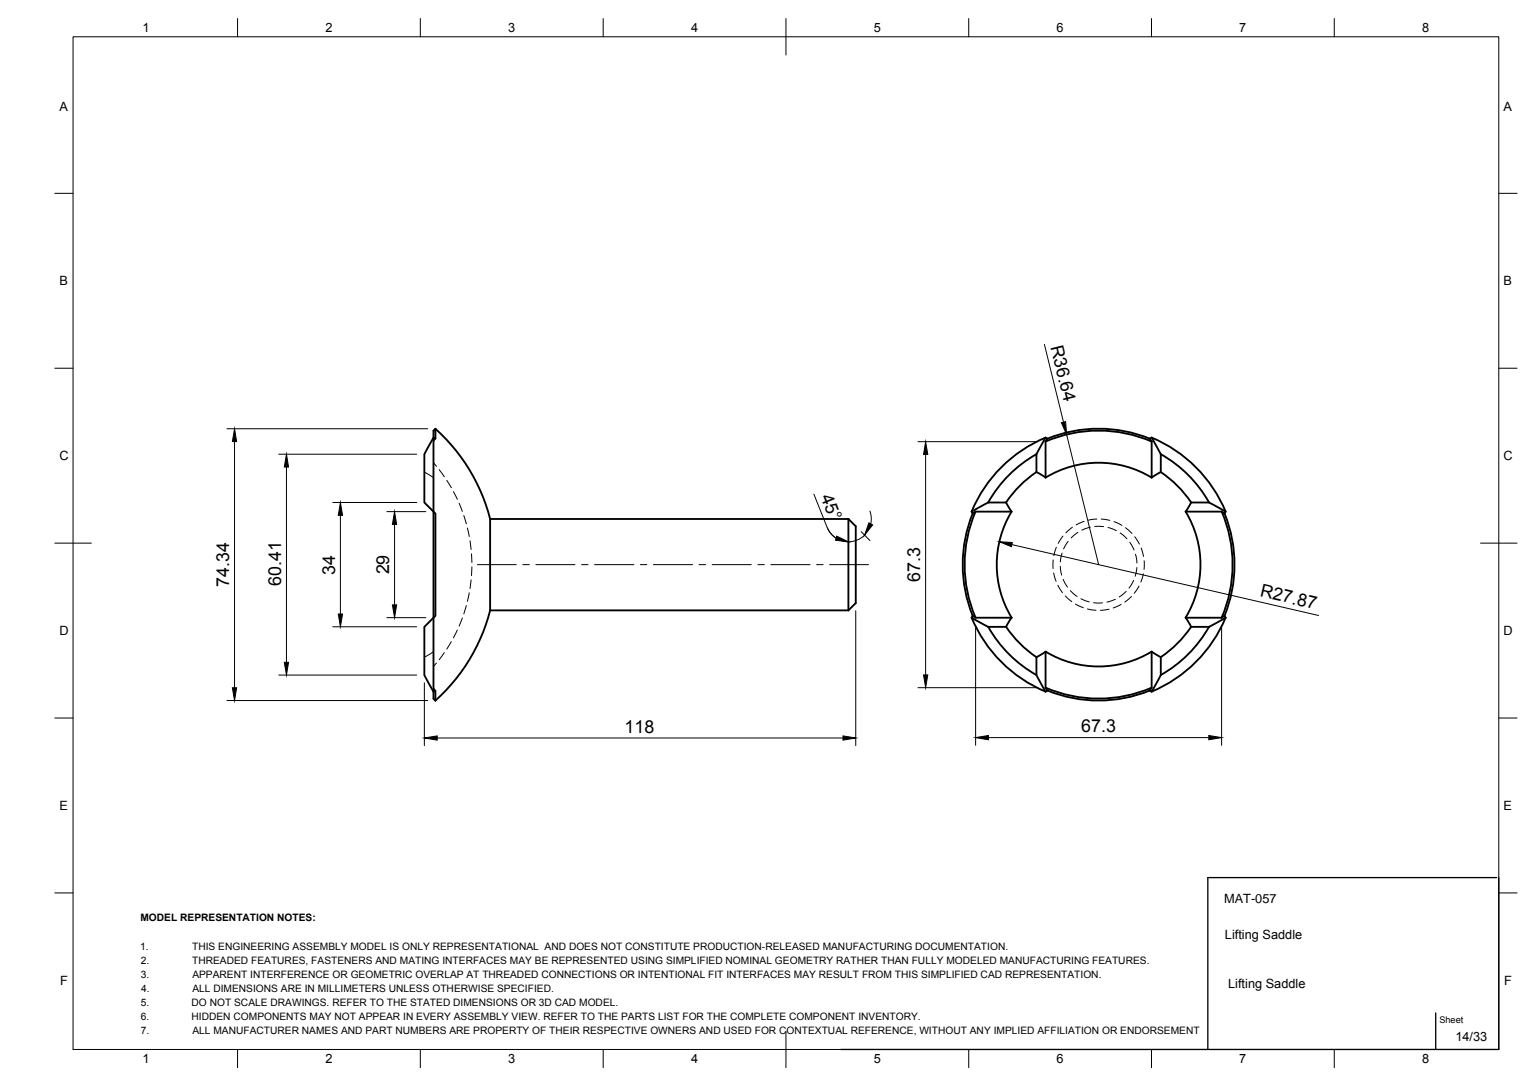
ISO-10303-21;
HEADER;
/* Generated by software containing ST-Developer
 * from STEP Tools, Inc. (www.steptools.com) 
 */

FILE_DESCRIPTION(
/* description */ ('STEP AP214', 'CAx-IF Rec.Pracs.---Representation and Presentation of Product Manufa
cturing Information (PMI)---4.0---2014-10-13'),
/* implementation_level */ '2;1');

FILE_NAME(
/* name */ 'Lifting Saddle.step',
/* time_stamp */ '2026-10-28T23:34:22+01:00',
/* author */ (''),
/* organization */ (''),
/* preprocessor_version */ 'ST-DEVELOPER v20.2',
/* originating_system */ 'Autodesk Translation Framework v15.17.0.0',
/* authorisation */ '');

FILE_SCHEMA (('AP242_MANAGED_MODEL_BASED_3D_ENGINEERING_MIM_LF { 1 0 10303 442 2 1 4 }'));
ENDSEC;

DATA;
#10=MECHANICAL_DESIGN_GEOMETRIC_PRESENTATION_REPRESENTATION('',(#254),#27807);
#19=(
BOUNDED_CURVE()
B_SPLINE_CURVE(2,(#18866,#18867,#18868),.UNSPECIFIED.,.F.,.F.)
B_SPLINE_CURVE_WITH_KNOTS((3,3),(0.462320796050368,0.567966350815043),
 .UNSPECIFIED.)
CURVE()
GEOMETRIC_REPRESENTATION_ITEM()
RATIONAL_B_SPLINE_CURVE((1.,1.,1.))
REPRESENTATION_ITEM('')
);
#20=(
BOUNDED_CURVE()
B_SPLINE_CURVE(2,(#18871,#18872,#18873),.UNSPECIFIED.,.F.,.F.)
B_SPLINE_CURVE_WITH_KNOTS((3,3),(-0.506850088621986,-0.399941526123303),
 .UNSPECIFIED.)
CURVE()
GEOMETRIC_REPRESENTATION_ITEM()
RATIONAL_B_SPLINE_CURVE((1.,1.,1.))
REPRESENTATION_ITEM('')
);
#21=(
BOUNDED_CURVE()
B_SPLINE_CURVE(2,(#18943,#18944,#18945),.UNSPECIFIED.,.F.,.F.)
B_SPLINE_CURVE_WITH_KNOTS((3,3),(-1.16469188019449,-0.591849614034338),
 .UNSPECIFIED.)
CURVE()
GEOMETRIC_REPRESENTATION_ITEM()
RATIONAL_B_SPLINE_CURVE((1.00111192291213,1.0014724056847,1.00120930695841))
REPRESENTATION_ITEM('')
);
#22=(
BOUNDED_CURVE()
B_SPLINE_CURVE(2,(#18948,#18949,#18950),.UNSPECIFIED.,.F.,.F.)
B_SPLINE_CURVE_WITH_KNOTS((3,3),(-1.18185454921906,-0.605722145160145),
 .UNSPECIFIED.)
CURVE()
GEOMETRIC_REPRESENTATION_ITEM()
RATIONAL_B_SPLINE_CURVE((1.00132604672167,1.00164254091047,1.00133534531621))
REPRESENTATION_ITEM('')
);
#23=(
BOUNDED_CURVE()
B_SPLINE_CURVE(2,(#18953,#18954,#18955),.UNSPECIFIED.,.F.,.F.)
B_SPLINE_CURVE_WITH_KNOTS((3,3),(-0.946143001046764,-0.369969297191779),
 .UNSPECIFIED.)
CURVE()
GEOMETRIC_REPRESENTATION_ITEM()
RATIONAL_B_SPLINE_CURVE((1.00070944583239,1.00100518872376,1.00067763892158))
REPRESENTATION_ITEM('')
);
#24=(
BOUNDED_CURVE()
B_SPLINE_CURVE(2,(#18958,#18959,#18960),.UNSPECIFIED.,.F.,.F.)
B_SPLINE_CURVE_WITH_KNOTS((3,3),(-0.972871322664165,-0.396853569144702),
 .UNSPECIFIED.)
CURVE()
GEOMETRIC_REPRESENTATION_ITEM()
RATIONAL_B_SPLINE_CURVE((1.00068050124441,1.00100540421751,1.00070701428562))
REPRESENTATION_ITEM('')
);
#25=(
BOUNDED_CURVE()
B_SPLINE_CURVE(2,(#18963,#18964,#18965),.UNSPECIFIED.,.F.,.F.)
B_SPLINE_CURVE_WITH_KNOTS((3,3),(-0.941872789970313,-0.366965630408099),
 .UNSPECIFIED.)
CURVE()
GEOMETRIC_REPRESENTATION_ITEM()
RATIONAL_B_SPLINE_CURVE((1.00063627989739,1.00095263621267,1.00064573232675))
REPRESENTATION_ITEM('')
);
#26=(
BOUNDED_CURVE()
B_SPLINE_CURVE(2,(#18968,#18969,#18970),.UNSPECIFIED.,.F.,.F.)
B_SPLINE_CURVE_WITH_KNOTS((3,3),(-0.937693085710887,-0.362724124749258),
 .UNSPECIFIED.)
CURVE()
GEOMETRIC_REPRESENTATION_ITEM()
RATIONAL_B_SPLINE_CURVE((1.00065371087358,1.00096152079163,1.00064606496848))
REPRESENTATION_ITEM('')
);
#27=(
BOUNDED_CURVE()
B_SPLINE_CURVE(2,(#18974,#18975,#18976),.UNSPECIFIED.,.F.,.F.)
B_SPLINE_CURVE_WITH_KNOTS((3,3),(-1.17291409885218,-0.596764361726987),
 .UNSPECIFIED.)
CURVE()
GEOMETRIC_REPRESENTATION_ITEM()
RATIONAL_B_SPLINE_CURVE((1.00133527889567,1.00164217359151,1.00132537873593))
REPRESENTATION_ITEM('')
);
#28=(
BOUNDED_CURVE()
B_SPLINE_CURVE(2,(#18979,#18980,#18981),.UNSPECIFIED.,.F.,.F.)
B_SPLINE_CURVE_WITH_KNOTS((3,3),(-1.0750860439484,-0.50223001899858),
 .UNSPECIFIED.)
CURVE()
GEOMETRIC_REPRESENTATION_ITEM()
RATIONAL_B_SPLINE_CURVE((1.00120779728153,1.00147115277612,1.00111092752705))
REPRESENTATION_ITEM('')
);
#29=(
BOUNDED_CURVE()
B_SPLINE_CURVE(2,(#18990,#18991,#18992),.UNSPECIFIED.,.F.,.F.)
B_SPLINE_CURVE_WITH_KNOTS((3,3),(0.837657703679305,0.944563738178637),
 .UNSPECIFIED.)
CURVE()
GEOMETRIC_REPRESENTATION_ITEM()
RATIONAL_B_SPLINE_CURVE((1.,1.,1.))
REPRESENTATION_ITEM('')
);
#30=(
BOUNDED_CURVE()
B_SPLINE_CURVE(2,(#18995,#18996,#18997),.UNSPECIFIED.,.F.,.F.)
B_SPLINE_CURVE_WITH_KNOTS((3,3),(0.387236418043007,0.493098305093553),
 .UNSPECIFIED.)
CURVE()
GEOMETRIC_REPRESENTATION_ITEM()
RATIONAL_B_SPLINE_CURVE((1.,1.,1.))
REPRESENTATION_ITEM('')
);
#31=(
BOUNDED_CURVE()
B_SPLINE_CURVE(2,(#19002,#19003,#19004),.UNSPECIFIED.,.F.,.F.)
B_SPLINE_CURVE_WITH_KNOTS((3,3),(1.14286008392437,1.24851586608623),
 .UNSPECIFIED.)
CURVE()
GEOMETRIC_REPRESENTATION_ITEM()
RATIONAL_B_SPLINE_CURVE((1.,1.,1.))
REPRESENTATION_ITEM('')
);
#32=(
BOUNDED_CURVE()
B_SPLINE_CURVE(2,(#19008,#19009,#19010),.UNSPECIFIED.,.F.,.F.)
B_SPLINE_CURVE_WITH_KNOTS((3,3),(0.394209164646282,0.501069286795388),
 .UNSPECIFIED.)
CURVE()
GEOMETRIC_REPRESENTATION_ITEM()
RATIONAL_B_SPLINE_CURVE((1.,1.,1.))
REPRESENTATION_ITEM('')
);
#33=(
BOUNDED_CURVE()
B_SPLINE_CURVE(2,(#19024,#19025,#19026),.UNSPECIFIED.,.F.,.F.)
B_SPLINE_CURVE_WITH_KNOTS((3,3),(0.39176954416594,0.498714042529527),
 .UNSPECIFIED.)
CURVE()
GEOMETRIC_REPRESENTATION_ITEM()
RATIONAL_B_SPLINE_CURVE((1.,1.,1.))
REPRESENTATION_ITEM('')
);
#34=(
BOUNDED_CURVE()
B_SPLINE_CURVE(2,(#19032,#19033,#19034),.UNSPECIFIED.,.F.,.F.)
B_SPLINE_CURVE_WITH_KNOTS((3,3),(1.0400161958356,1.14585618521608),
 .UNSPECIFIED.)
CURVE()
GEOMETRIC_REPRESENTATION_ITEM()
RATIONAL_B_SPLINE_CURVE((1.,1.,1.))
REPRESENTATION_ITEM('')
);
#209=SHAPE_REPRESENTATION_RELATIONSHIP('SRR','None',#27905,#231);
#231=ADVANCED_BREP_SHAPE_REPRESENTATION('',(#283),#27785);
#254=STYLED_ITEM('',(#28070),#283);
#283=MANIFOLD_SOLID_BREP('Body1',#12030);
#329=SPHERICAL_SURFACE('',#12793,42.2295496985778);
#330=SPHERICAL_SURFACE('',#12810,50.);
#377=FACE_BOUND('',#2215,.T.);
#542=PLANE('',#12834);
#543=PLANE('',#12837);
#544=PLANE('',#12839);
#545=PLANE('',#12840);
#546=PLANE('',#12841);
#547=PLANE('',#12842);
#548=PLANE('',#12843);
#549=PLANE('',#12845);
#550=PLANE('',#12846);
#551=PLANE('',#12847);
#552=PLANE('',#12848);
#553=PLANE('',#12849);
#554=PLANE('',#12850);
#555=PLANE('',#12852);
#556=PLANE('',#12853);
#557=PLANE('',#12854);
#558=PLANE('',#12855);
#1072=CYLINDRICAL_SURFACE('',#12827,12.5);
#1472=FACE_OUTER_BOUND('',#2211,.T.);
#1473=FACE_OUTER_BOUND('',#2212,.T.);
#1474=FACE_OUTER_BOUND('',#2213,.T.);
#1475=FACE_OUTER_BOUND('',#2214,.T.);
#1476=FACE_OUTER_BOUND('',#2216,.T.);
#1477=FACE_OUTER_BOUND('',#2217,.T.);
#1478=FACE_OUTER_BOUND('',#2218,.T.);
#1479=FACE_OUTER_BOUND('',#2219,.T.);
#1480=FACE_OUTER_BOUND('',#2220,.T.);
#1481=FACE_OUTER_BOUND('',#2221,.T.);
#1482=FACE_OUTER_BOUND('',#2222,.T.);
#1483=FACE_OUTER_BOUND('',#2223,.T.);
#1484=FACE_OUTER_BOUND('',#2224,.T.);
#1485=FACE_OUTER_BOUND('',#2225,.T.);
#1486=FACE_OUTER_BOUND('',#2226,.T.);
#1487=FACE_OUTER_BOUND('',#2227,.T.);
#1488=FACE_OUTER_BOUND('',#2228,.T.);
#1489=FACE_OUTER_BOUND('',#2229,.T.);
#1490=FACE_OUTER_BOUND('',#2230,.T.);
#1491=FACE_OUTER_BOUND('',#2231,.T.);
#1492=FACE_OUTER_BOUND('',#2232,.T.);
#1493=FACE_OUTER_BOUND('',#2233,.T.);
#1494=FACE_OUTER_BOUND('',#2234,.T.);
#1495=FACE_OUTER_BOUND('',#2235,.T.);
#1496=FACE_OUTER_BOUND('',#2236,.T.);
#1497=FACE_OUTER_BOUND('',#2237,.T.);
#1498=FACE_OUTER_BOUND('',#2238,.T.);
#1499=FACE_OUTER_BOUND('',#2239,.T.);
#1500=FACE_OUTER_BOUND('',#2240,.T.);
#2211=EDGE_LOOP('',(#9013,#9014,#9015,#9016,#9017));
#2212=EDGE_LOOP('',(#9018,#9019,#9020,#9021));
#2213=EDGE_LOOP('',(#9022,#9023,#9024,#9025,#9026,#9027,#9028,#9029,#9030,
#9031,#9032,#9033,#9034,#9035,#9036,#9037));
#2214=EDGE_LOOP('',(#9038,#9039,#9040,#9041,#9042,#9043,#9044,#9045,#9046,
#9047,#9048,#9049,#9050,#9051,#9052,#9053));
#2215=EDGE_LOOP('',(#9054));
#2216=EDGE_LOOP('',(#9055,#9056,#9057,#9058,#9059));
#2217=EDGE_LOOP('',(#9060,#9061,#9062,#9063));
#2218=EDGE_LOOP('',(#9064,#9065,#9066,#9067));
#2219=EDGE_LOOP('',(#9068,#9069,#9070,#9071));
#2220=EDGE_LOOP('',(#9072));
#2221=EDGE_LOOP('',(#9073,#9074,#9075,#9076));
#2222=EDGE_LOOP('',(#9077,#9078,#9079,#9080));
#2223=EDGE_LOOP('',(#9081,#9082,#9083,#9084,#9085,#9086));
#2224=EDGE_LOOP('',(#9087,#9088,#9089,#9090,#9091,#9092));
#2225=EDGE_LOOP('',(#9093,#9094,#9095,#9096,#9097,#9098));
#2226=EDGE_LOOP('',(#9099,#9100,#9101,#9102,#9103,#9104));
#2227=EDGE_LOOP('',(#9105,#9106,#9107,#9108));
#2228=EDGE_LOOP('',(#9109,#9110,#9111,#9112));
#2229=EDGE_LOOP('',(#9113,#9114,#9115,#9116,#9117,#9118));
#2230=EDGE_LOOP('',(#9119,#9120,#9121,#9122,#9123,#9124));
#2231=EDGE_LOOP('',(#9125,#9126,#9127,#9128,#9129,#9130));
#2232=EDGE_LOOP('',(#9131,#9132,#9133,#9134,#9135,#9136));
#2233=EDGE_LOOP('',(#9137,#9138,#9139,#9140));
#2234=EDGE_LOOP('',(#9141,#9142,#9143,#9144));
#2235=EDGE_LOOP('',(#9145,#9146,#9147,#9148));
#2236=EDGE_LOOP('',(#9149,#9150,#9151,#9152));
#2237=EDGE_LOOP('',(#9153,#9154,#9155,#9156));
#2238=EDGE_LOOP('',(#9157,#9158,#9159,#9160));
#2239=EDGE_LOOP('',(#9161,#9162,#9163,#9164));
#2240=EDGE_LOOP('',(#9165,#9166,#9167,#9168));
#3055=LINE('',#18859,#3875);
#3056=LINE('',#18940,#3876);
#3057=LINE('',#18984,#3877);
#3058=LINE('',#18987,#3878);
#3059=LINE('',#18989,#3879);
#3060=LINE('',#18994,#3880);
#3061=LINE('',#18999,#3881);
#3062=LINE('',#19001,#3882);
#3063=LINE('',#19006,#3883);
#3064=LINE('',#19011,#3884);
#3065=LINE('',#19015,#3885);
#3066=LINE('',#19016,#3886);
#3067=LINE('',#19018,#3887);
#3068=LINE('',#19020,#3888);
#3069=LINE('',#19022,#3889);
#3070=LINE('',#19027,#3890);
#3071=LINE('',#19029,#3891);
#3072=LINE('',#19031,#3892);
#3875=VECTOR('',#15015,10.5);
#3876=VECTOR('',#15094,12.5);
#3877=VECTOR('',#15115,1000.);
#3878=VECTOR('',#15118,1000.);
#3879=VECTOR('',#15121,1000.);
#3880=VECTOR('',#15124,1000.);
#3881=VECTOR('',#15127,1000.);
#3882=VECTOR('',#15128,1000.);
#3883=VECTOR('',#15131,1000.);
#3884=VECTOR('',#15132,1000.);
#3885=VECTOR('',#15139,1000.);
#3886=VECTOR('',#15140,1000.);
#3887=VECTOR('',#15143,1000.);
#3888=VECTOR('',#15146,1000.);
#3889=VECTOR('',#15149,1000.);
#3890=VECTOR('',#15150,1000.);
#3891=VECTOR('',#15153,1000.);
#3892=VECTOR('',#15154,1000.);
#4625=CIRCLE('',#12787,12.5);
#4626=CIRCLE('',#12788,12.5);
#4627=CIRCLE('',#12789,10.5);
#4628=CIRCLE('',#12791,36.6405776438474);
#4629=CIRCLE('',#12792,37.1705339516543);
#4630=CIRCLE('',#12794,27.867569521218);
#4631=CIRCLE('',#12795,26.7352152856439);
#4632=CIRCLE('',#12796,30.4789811536249);
#4633=CIRCLE('',#12797,26.7352152856439);
#4634=CIRCLE('',#12798,27.867569521218);
#4635=CIRCLE('',#12799,26.7352152856438);
#4636=CIRCLE('',#12800,30.4789811536249);
#4637=CIRCLE('',#12801,26.7352152856439);
#4638=CIRCLE('',#12802,27.867569521218);
#4639=CIRCLE('',#12803,26.7352152856439);
#4640=CIRCLE('',#12804,30.4789811536249);
#4641=CIRCLE('',#12805,26.7352152856439);
#4642=CIRCLE('',#12806,27.867569521218);
#4643=CIRCLE('',#12807,26.7352152856439);
#4644=CIRCLE('',#12808,30.4789811536249);
#4645=CIRCLE('',#12809,26.7352152856439);
#4646=CIRCLE('',#12811,37.1705339516543);
#4647=CIRCLE('',#12812,37.0952876899206);
#4648=CIRCLE('',#12813,37.6405776438474);
#4649=CIRCLE('',#12814,37.0952876899207);
#4650=CIRCLE('',#12815,37.0952876899206);
#4651=CIRCLE('',#12816,37.6405776438474);
#4652=CIRCLE('',#12817,37.0952876899206);
#4653=CIRCLE('',#12818,37.1705339516542);
#4654=CIRCLE('',#12819,37.0952876899206);
#4655=CIRCLE('',#12820,37.6405776438474);
#4656=CIRCLE('',#12821,37.0952876899206);
#4657=CIRCLE('',#12822,37.1705339516543);
#4658=CIRCLE('',#12823,37.0952876899207);
#4659=CIRCLE('',#12824,37.6405776438474);
#4660=CIRCLE('',#12825,37.0952876899206);
#4661=CIRCLE('',#12826,12.5);
#4662=CIRCLE('',#12829,34.6617737272029);
#4663=CIRCLE('',#12831,34.6617737272029);
#4664=CIRCLE('',#12833,34.6617737272029);
#4665=CIRCLE('',#12836,34.6617737272029);
#4666=CIRCLE('',#12838,36.6405776438474);
#4667=CIRCLE('',#12844,36.6405776438474);
#4668=CIRCLE('',#12851,36.6405776438474);
#5409=VERTEX_POINT('',#18854);
#5410=VERTEX_POINT('',#18855);
#5411=VERTEX_POINT('',#18858);
#5412=VERTEX_POINT('',#18862);
#5413=VERTEX_POINT('',#18863);
#5414=VERTEX_POINT('',#18865);
#5415=VERTEX_POINT('',#18869);
#5416=VERTEX_POINT('',#18875);
#5417=VERTEX_POINT('',#18876);
#5418=VERTEX_POINT('',#18878);
#5419=VERTEX_POINT('',#18880);
#5420=VERTEX_POINT('',#18882);
#5421=VERTEX_POINT('',#18884);
#5422=VERTEX_POINT('',#18886);
#5423=VERTEX_POINT('',#18888);
#5424=VERTEX_POINT('',#18890);
#5425=VERTEX_POINT('',#18892);
#5426=VERTEX_POINT('',#18894);
#5427=VERTEX_POINT('',#18896);
#5428=VERTEX_POINT('',#18898);
#5429=VERTEX_POINT('',#18900);
#5430=VERTEX_POINT('',#18902);
#5431=VERTEX_POINT('',#18904);
#5432=VERTEX_POINT('',#18908);
#5433=VERTEX_POINT('',#18909);
#5434=VERTEX_POINT('',#18911);
#5435=VERTEX_POINT('',#18913);
#5436=VERTEX_POINT('',#18916);
#5437=VERTEX_POINT('',#18918);
#5438=VERTEX_POINT('',#18920);
#5439=VERTEX_POINT('',#18922);
#5440=VERTEX_POINT('',#18924);
#5441=VERTEX_POINT('',#18926);
#5442=VERTEX_POINT('',#18928);
#5443=VERTEX_POINT('',#18930);
#5444=VERTEX_POINT('',#18932);
#5445=VERTEX_POINT('',#18934);
#5446=VERTEX_POINT('',#18937);
#5447=VERTEX_POINT('',#18942);
#5448=VERTEX_POINT('',#18946);
#5449=VERTEX_POINT('',#18952);
#5450=VERTEX_POINT('',#18956);
#5451=VERTEX_POINT('',#18962);
#5452=VERTEX_POINT('',#18966);
#5453=VERTEX_POINT('',#18973);
#5454=VERTEX_POINT('',#18977);
#5455=VERTEX_POINT('',#18983);
#5456=VERTEX_POINT('',#18985);
#5457=VERTEX_POINT('',#19000);
#5458=VERTEX_POINT('',#19007);
#5459=VERTEX_POINT('',#19023);
#5460=VERTEX_POINT('',#19030);
#6719=EDGE_CURVE('',#5409,#5410,#4625,.T.);
#6720=EDGE_CURVE('',#5410,#5409,#4626,.T.);
#6721=EDGE_CURVE('',#5410,#5411,#3055,.T.);
#6722=EDGE_CURVE('',#5411,#5411,#4627,.T.);
#6723=EDGE_CURVE('',#5412,#5413,#4628,.T.);
#6724=EDGE_CURVE('',#5414,#5412,#19,.T.);
#6725=EDGE_CURVE('',#5415,#5414,#4629,.T.);
#6726=EDGE_CURVE('',#5413,#5415,#20,.T.);
#6727=EDGE_CURVE('',#5416,#5417,#4630,.T.);
#6728=EDGE_CURVE('',#5417,#5418,#4631,.T.);
#6729=EDGE_CURVE('',#5418,#5419,#4632,.T.);
#6730=EDGE_CURVE('',#5419,#5420,#4633,.T.);
#6731=EDGE_CURVE('',#5420,#5421,#4634,.T.);
#6732=EDGE_CURVE('',#5421,#5422,#4635,.T.);
#6733=EDGE_CURVE('',#5422,#5423,#4636,.T.);
#6734=EDGE_CURVE('',#5423,#5424,#4637,.T.);
#6735=EDGE_CURVE('',#5424,#5425,#4638,.T.);
#6736=EDGE_CURVE('',#5425,#5426,#4639,.T.);
#6737=EDGE_CURVE('',#5426,#5427,#4640,.T.);
#6738=EDGE_CURVE('',#5427,#5428,#4641,.T.);
#6739=EDGE_CURVE('',#5428,#5429,#4642,.T.);
#6740=EDGE_CURVE('',#5429,#5430,#4643,.T.);
#6741=EDGE_CURVE('',#5430,#5431,#4644,.T.);
#6742=EDGE_CURVE('',#5431,#5416,#4645,.T.);
#6743=EDGE_CURVE('',#5432,#5433,#4646,.T.);
#6744=EDGE_CURVE('',#5433,#5434,#4647,.T.);
#6745=EDGE_CURVE('',#5434,#5435,#4648,.T.);
#6746=EDGE_CURVE('',#5435,#5415,#4649,.T.);
#6747=EDGE_CURVE('',#5414,#5436,#4650,.T.);
#6748=EDGE_CURVE('',#5436,#5437,#4651,.T.);
#6749=EDGE_CURVE('',#5437,#5438,#4652,.T.);
#6750=EDGE_CURVE('',#5438,#5439,#4653,.T.);
#6751=EDGE_CURVE('',#5439,#5440,#4654,.T.);
#6752=EDGE_CURVE('',#5440,#5441,#4655,.T.);
#6753=EDGE_CURVE('',#5441,#5442,#4656,.T.);
#6754=EDGE_CURVE('',#5442,#5443,#4657,.T.);
#6755=EDGE_CURVE('',#5443,#5444,#4658,.T.);
#6756=EDGE_CURVE('',#5444,#5445,#4659,.T.);
#6757=EDGE_CURVE('',#5445,#5432,#4660,.T.);
#6758=EDGE_CURVE('',#5446,#5446,#4661,.T.);
#6759=EDGE_CURVE('',#5409,#5446,#3056,.T.);
#6760=EDGE_CURVE('',#5444,#5447,#21,.T.);
#6761=EDGE_CURVE('',#5447,#5448,#4662,.T.);
#6762=EDGE_CURVE('',#5448,#5445,#22,.T.);
#6763=EDGE_CURVE('',#5434,#5449,#23,.T.);
#6764=EDGE_CURVE('',#5449,#5450,#4663,.T.);
#6765=EDGE_CURVE('',#5450,#5435,#24,.T.);
#6766=EDGE_CURVE('',#5440,#5451,#25,.T.);
#6767=EDGE_CURVE('',#5451,#5452,#4664,.T.);
#6768=EDGE_CURVE('',#5452,#5441,#26,.T.);
#6769=EDGE_CURVE('',#5436,#5453,#27,.T.);
#6770=EDGE_CURVE('',#5453,#5454,#4665,.T.);
#6771=EDGE_CURVE('',#5454,#5437,#28,.T.);
#6772=EDGE_CURVE('',#5424,#5455,#3057,.T.);
#6773=EDGE_CURVE('',#5455,#5456,#4666,.T.);
#6774=EDGE_CURVE('',#5425,#5456,#3058,.T.);
#6775=EDGE_CURVE('',#5454,#5426,#3059,.T.);
#6776=EDGE_CURVE('',#5456,#5438,#29,.T.);
#6777=EDGE_CURVE('',#5423,#5451,#3060,.T.);
#6778=EDGE_CURVE('',#5439,#5455,#30,.T.);
#6779=EDGE_CURVE('',#5448,#5418,#3061,.T.);
#6780=EDGE_CURVE('',#5457,#5417,#3062,.T.);
#6781=EDGE_CURVE('',#5457,#5432,#31,.T.);
#6782=EDGE_CURVE('',#5431,#5449,#3063,.T.);
#6783=EDGE_CURVE('',#5433,#5458,#32,.T.);
#6784=EDGE_CURVE('',#5458,#5416,#3064,.T.);
#6785=EDGE_CURVE('',#5458,#5457,#4667,.T.);
#6786=EDGE_CURVE('',#5412,#5428,#3065,.T.);
#6787=EDGE_CURVE('',#5413,#5429,#3066,.T.);
#6788=EDGE_CURVE('',#5427,#5453,#3067,.T.);
#6789=EDGE_CURVE('',#5450,#5430,#3068,.T.);
#6790=EDGE_CURVE('',#5419,#5447,#3069,.T.);
#6791=EDGE_CURVE('',#5443,#5459,#33,.T.);
#6792=EDGE_CURVE('',#5420,#5459,#3070,.T.);
#6793=EDGE_CURVE('',#5452,#5422,#3071,.T.);
#6794=EDGE_CURVE('',#5421,#5460,#3072,.T.);
#6795=EDGE_CURVE('',#5460,#5442,#34,.T.);
#6796=EDGE_CURVE('',#5459,#5460,#4668,.T.);
#9013=ORIENTED_EDGE('',*,*,#6719,.F.);
#9014=ORIENTED_EDGE('',*,*,#6720,.F.);
#9015=ORIENTED_EDGE('',*,*,#6721,.T.);
#9016=ORIENTED_EDGE('',*,*,#6722,.F.);
#9017=ORIENTED_EDGE('',*,*,#6721,.F.);
#9018=ORIENTED_EDGE('',*,*,#6723,.F.);
#9019=ORIENTED_EDGE('',*,*,#6724,.F.);
#9020=ORIENTED_EDGE('',*,*,#6725,.F.);
#9021=ORIENTED_EDGE('',*,*,#6726,.F.);
#9022=ORIENTED_EDGE('',*,*,#6727,.T.);
#9023=ORIENTED_EDGE('',*,*,#6728,.T.);
#9024=ORIENTED_EDGE('',*,*,#6729,.T.);
#9025=ORIENTED_EDGE('',*,*,#6730,.T.);
#9026=ORIENTED_EDGE('',*,*,#6731,.T.);
#9027=ORIENTED_EDGE('',*,*,#6732,.T.);
#9028=ORIENTED_EDGE('',*,*,#6733,.T.);
#9029=ORIENTED_EDGE('',*,*,#6734,.T.);
#9030=ORIENTED_EDGE('',*,*,#6735,.T.);
#9031=ORIENTED_EDGE('',*,*,#6736,.T.);
#9032=ORIENTED_EDGE('',*,*,#6737,.T.);
#9033=ORIENTED_EDGE('',*,*,#6738,.T.);
#9034=ORIENTED_EDGE('',*,*,#6739,.T.);
#9035=ORIENTED_EDGE('',*,*,#6740,.T.);
#9036=ORIENTED_EDGE('',*,*,#6741,.T.);
#9037=ORIENTED_EDGE('',*,*,#6742,.T.);
#9038=ORIENTED_EDGE('',*,*,#6743,.T.);
#9039=ORIENTED_EDGE('',*,*,#6744,.T.);
#9040=ORIENTED_EDGE('',*,*,#6745,.T.);
#9041=ORIENTED_EDGE('',*,*,#6746,.T.);
#9042=ORIENTED_EDGE('',*,*,#6725,.T.);
#9043=ORIENTED_EDGE('',*,*,#6747,.T.);
#9044=ORIENTED_EDGE('',*,*,#6748,.T.);
#9045=ORIENTED_EDGE('',*,*,#6749,.T.);
#9046=ORIENTED_EDGE('',*,*,#6750,.T.);
#9047=ORIENTED_EDGE('',*,*,#6751,.T.);
#9048=ORIENTED_EDGE('',*,*,#6752,.T.);
#9049=ORIENTED_EDGE('',*,*,#6753,.T.);
#9050=ORIENTED_EDGE('',*,*,#6754,.T.);
#9051=ORIENTED_EDGE('',*,*,#6755,.T.);
#9052=ORIENTED_EDGE('',*,*,#6756,.T.);
#9053=ORIENTED_EDGE('',*,*,#6757,.T.);
#9054=ORIENTED_EDGE('',*,*,#6758,.F.);
#9055=ORIENTED_EDGE('',*,*,#6719,.T.);
#9056=ORIENTED_EDGE('',*,*,#6720,.T.);
#9057=ORIENTED_EDGE('',*,*,#6759,.T.);
#9058=ORIENTED_EDGE('',*,*,#6758,.T.);
#9059=ORIENTED_EDGE('',*,*,#6759,.F.);
#9060=ORIENTED_EDGE('',*,*,#6760,.T.);
#9061=ORIENTED_EDGE('',*,*,#6761,.T.);
#9062=ORIENTED_EDGE('',*,*,#6762,.T.);
#9063=ORIENTED_EDGE('',*,*,#6756,.F.);
#9064=ORIENTED_EDGE('',*,*,#6763,.T.);
#9065=ORIENTED_EDGE('',*,*,#6764,.T.);
#9066=ORIENTED_EDGE('',*,*,#6765,.T.);
#9067=ORIENTED_EDGE('',*,*,#6745,.F.);
#9068=ORIENTED_EDGE('',*,*,#6766,.T.);
#9069=ORIENTED_EDGE('',*,*,#6767,.T.);
#9070=ORIENTED_EDGE('',*,*,#6768,.T.);
#9071=ORIENTED_EDGE('',*,*,#6752,.F.);
#9072=ORIENTED_EDGE('',*,*,#6722,.T.);
#9073=ORIENTED_EDGE('',*,*,#6769,.T.);
#9074=ORIENTED_EDGE('',*,*,#6770,.T.);
#9075=ORIENTED_EDGE('',*,*,#6771,.T.);
#9076=ORIENTED_EDGE('',*,*,#6748,.F.);
#9077=ORIENTED_EDGE('',*,*,#6772,.T.);
#9078=ORIENTED_EDGE('',*,*,#6773,.T.);
#9079=ORIENTED_EDGE('',*,*,#6774,.F.);
#9080=ORIENTED_EDGE('',*,*,#6735,.F.);
#9081=ORIENTED_EDGE('',*,*,#6771,.F.);
#9082=ORIENTED_EDGE('',*,*,#6775,.T.);
#9083=ORIENTED_EDGE('',*,*,#6736,.F.);
#9084=ORIENTED_EDGE('',*,*,#6774,.T.);
#9085=ORIENTED_EDGE('',*,*,#6776,.T.);
#9086=ORIENTED_EDGE('',*,*,#6749,.F.);
#9087=ORIENTED_EDGE('',*,*,#6734,.F.);
#9088=ORIENTED_EDGE('',*,*,#6777,.T.);
#9089=ORIENTED_EDGE('',*,*,#6766,.F.);
#9090=ORIENTED_EDGE('',*,*,#6751,.F.);
#9091=ORIENTED_EDGE('',*,*,#6778,.T.);
#9092=ORIENTED_EDGE('',*,*,#6772,.F.);
#9093=ORIENTED_EDGE('',*,*,#6762,.F.);
#9094=ORIENTED_EDGE('',*,*,#6779,.T.);
#9095=ORIENTED_EDGE('',*,*,#6728,.F.);
#9096=ORIENTED_EDGE('',*,*,#6780,.F.);
#9097=ORIENTED_EDGE('',*,*,#6781,.T.);
#9098=ORIENTED_EDGE('',*,*,#6757,.F.);
#9099=ORIENTED_EDGE('',*,*,#6742,.F.);
#9100=ORIENTED_EDGE('',*,*,#6782,.T.);
#9101=ORIENTED_EDGE('',*,*,#6763,.F.);
#9102=ORIENTED_EDGE('',*,*,#6744,.F.);
#9103=ORIENTED_EDGE('',*,*,#6783,.T.);
#9104=ORIENTED_EDGE('',*,*,#6784,.T.);
#9105=ORIENTED_EDGE('',*,*,#6784,.F.);
#9106=ORIENTED_EDGE('',*,*,#6785,.T.);
#9107=ORIENTED_EDGE('',*,*,#6780,.T.);
#9108=ORIENTED_EDGE('',*,*,#6727,.F.);
#9109=ORIENTED_EDGE('',*,*,#6786,.F.);
#9110=ORIENTED_EDGE('',*,*,#6723,.T.);
#9111=ORIENTED_EDGE('',*,*,#6787,.T.);
#9112=ORIENTED_EDGE('',*,*,#6739,.F.);
#9113=ORIENTED_EDGE('',*,*,#6738,.F.);
#9114=ORIENTED_EDGE('',*,*,#6788,.T.);
#9115=ORIENTED_EDGE('',*,*,#6769,.F.);
#9116=ORIENTED_EDGE('',*,*,#6747,.F.);
#9117=ORIENTED_EDGE('',*,*,#6724,.T.);
#9118=ORIENTED_EDGE('',*,*,#6786,.T.);
#9119=ORIENTED_EDGE('',*,*,#6765,.F.);
#9120=ORIENTED_EDGE('',*,*,#6789,.T.);
#9121=ORIENTED_EDGE('',*,*,#6740,.F.);
#9122=ORIENTED_EDGE('',*,*,#6787,.F.);
#9123=ORIENTED_EDGE('',*,*,#6726,.T.);
#9124=ORIENTED_EDGE('',*,*,#6746,.F.);
#9125=ORIENTED_EDGE('',*,*,#6730,.F.);
#9126=ORIENTED_EDGE('',*,*,#6790,.T.);
#9127=ORIENTED_EDGE('',*,*,#6760,.F.);
#9128=ORIENTED_EDGE('',*,*,#6755,.F.);
#9129=ORIENTED_EDGE('',*,*,#6791,.T.);
#9130=ORIENTED_EDGE('',*,*,#6792,.F.);
#9131=ORIENTED_EDGE('',*,*,#6768,.F.);
#9132=ORIENTED_EDGE('',*,*,#6793,.T.);
#9133=ORIENTED_EDGE('',*,*,#6732,.F.);
#9134=ORIENTED_EDGE('',*,*,#6794,.T.);
#9135=ORIENTED_EDGE('',*,*,#6795,.T.);
#9136=ORIENTED_EDGE('',*,*,#6753,.F.);
#9137=ORIENTED_EDGE('',*,*,#6792,.T.);
#9138=ORIENTED_EDGE('',*,*,#6796,.T.);
#9139=ORIENTED_EDGE('',*,*,#6794,.F.);
#9140=ORIENTED_EDGE('',*,*,#6731,.F.);
#9141=ORIENTED_EDGE('',*,*,#6733,.F.);
#9142=ORIENTED_EDGE('',*,*,#6793,.F.);
#9143=ORIENTED_EDGE('',*,*,#6767,.F.);
#9144=ORIENTED_EDGE('',*,*,#6777,.F.);
#9145=ORIENTED_EDGE('',*,*,#6761,.F.);
#9146=ORIENTED_EDGE('',*,*,#6790,.F.);
#9147=ORIENTED_EDGE('',*,*,#6729,.F.);
#9148=ORIENTED_EDGE('',*,*,#6779,.F.);
#9149=ORIENTED_EDGE('',*,*,#6741,.F.);
#9150=ORIENTED_EDGE('',*,*,#6789,.F.);
#9151=ORIENTED_EDGE('',*,*,#6764,.F.);
#9152=ORIENTED_EDGE('',*,*,#6782,.F.);
#9153=ORIENTED_EDGE('',*,*,#6770,.F.);
#9154=ORIENTED_EDGE('',*,*,#6788,.F.);
#9155=ORIENTED_EDGE('',*,*,#6737,.F.);
#9156=ORIENTED_EDGE('',*,*,#6775,.F.);
#9157=ORIENTED_EDGE('',*,*,#6776,.F.);
#9158=ORIENTED_EDGE('',*,*,#6773,.F.);
#9159=ORIENTED_EDGE('',*,*,#6778,.F.);
#9160=ORIENTED_EDGE('',*,*,#6750,.F.);
#9161=ORIENTED_EDGE('',*,*,#6795,.F.);
#9162=ORIENTED_EDGE('',*,*,#6796,.F.);
#9163=ORIENTED_EDGE('',*,*,#6791,.F.);
#9164=ORIENTED_EDGE('',*,*,#6754,.F.);
#9165=ORIENTED_EDGE('',*,*,#6781,.F.);
#9166=ORIENTED_EDGE('',*,*,#6785,.F.);
#9167=ORIENTED_EDGE('',*,*,#6783,.F.);
#9168=ORIENTED_EDGE('',*,*,#6743,.F.);
#11291=CONICAL_SURFACE('',#12786,10.5,0.785398163397448);
#11292=CONICAL_SURFACE('',#12790,37.1705339516543,0.785398163397448);
#11293=CONICAL_SURFACE('',#12828,32.2782665420145,0.872664625997169);
#11294=CONICAL_SURFACE('',#12830,32.2782665420145,0.872664625997169);
#11295=CONICAL_SURFACE('',#12832,32.2782665420145,0.872664625997169);
#11296=CONICAL_SURFACE('',#12835,32.2782665420145,0.872664625997169);
#11297=CONICAL_SURFACE('',#12856,37.1705339516543,0.785398163397448);
#11298=CONICAL_SURFACE('',#12857,37.1705339516543,0.785398163397448);
#11299=CONICAL_SURFACE('',#12858,37.1705339516543,0.785398163397448);
#11554=ADVANCED_FACE('',(#1472),#11291,.T.);
#11555=ADVANCED_FACE('',(#1473),#11292,.T.);
#11556=ADVANCED_FACE('',(#1474),#329,.F.);
#11557=ADVANCED_FACE('',(#1475,#377),#330,.T.);
#11558=ADVANCED_FACE('',(#1476),#1072,.T.);
#11559=ADVANCED_FACE('',(#1477),#11293,.T.);
#11560=ADVANCED_FACE('',(#1478),#11294,.T.);
#11561=ADVANCED_FACE('',(#1479),#11295,.T.);
#11562=ADVANCED_FACE('',(#1480),#542,.F.);
#11563=ADVANCED_FACE('',(#1481),#11296,.T.);
#11564=ADVANCED_FACE('',(#1482),#543,.F.);
#11565=ADVANCED_FACE('',(#1483),#544,.F.);
#11566=ADVANCED_FACE('',(#1484),#545,.F.);
#11567=ADVANCED_FACE('',(#1485),#546,.F.);
#11568=ADVANCED_FACE('',(#1486),#547,.F.);
#11569=ADVANCED_FACE('',(#1487),#548,.F.);
#11570=ADVANCED_FACE('',(#1488),#549,.F.);
#11571=ADVANCED_FACE('',(#1489),#550,.F.);
#11572=ADVANCED_FACE('',(#1490),#551,.F.);
#11573=ADVANCED_FACE('',(#1491),#552,.F.);
#11574=ADVANCED_FACE('',(#1492),#553,.F.);
#11575=ADVANCED_FACE('',(#1493),#554,.F.);
#11576=ADVANCED_FACE('',(#1494),#555,.F.);
#11577=ADVANCED_FACE('',(#1495),#556,.F.);
#11578=ADVANCED_FACE('',(#1496),#557,.F.);
#11579=ADVANCED_FACE('',(#1497),#558,.F.);
#11580=ADVANCED_FACE('',(#1498),#11297,.T.);
#11581=ADVANCED_FACE('',(#1499),#11298,.T.);
#11582=ADVANCED_FACE('',(#1500),#11299,.T.);
#12030=CLOSED_SHELL('',(#11554,#11555,#11556,#11557,#11558,#11559,#11560,
#11561,#11562,#11563,#11564,#11565,#11566,#11567,#11568,#11569,#11570,#11571,
#11572,#11573,#11574,#11575,#11576,#11577,#11578,#11579,#11580,#11581,#11582));
#12785=AXIS2_PLACEMENT_3D('',#18852,#15007,#15008);
#12786=AXIS2_PLACEMENT_3D('',#18853,#15009,#15010);
#12787=AXIS2_PLACEMENT_3D('',#18856,#15011,#15012);
#12788=AXIS2_PLACEMENT_3D('',#18857,#15013,#15014);
#12789=AXIS2_PLACEMENT_3D('',#18860,#15016,#15017);
#12790=AXIS2_PLACEMENT_3D('',#18861,#15018,#15019);
#12791=AXIS2_PLACEMENT_3D('',#18864,#15020,#15021);
#12792=AXIS2_PLACEMENT_3D('',#18870,#15022,#15023);
#12793=AXIS2_PLACEMENT_3D('',#18874,#15024,#15025);
#12794=AXIS2_PLACEMENT_3D('',#18877,#15026,#15027);
#12795=AXIS2_PLACEMENT_3D('',#18879,#15028,#15029);
#12796=AXIS2_PLACEMENT_3D('',#18881,#15030,#15031);
#12797=AXIS2_PLACEMENT_3D('',#18883,#15032,#15033);
#12798=AXIS2_PLACEMENT_3D('',#18885,#15034,#15035);
#12799=AXIS2_PLACEMENT_3D('',#18887,#15036,#15037);
#12800=AXIS2_PLACEMENT_3D('',#18889,#15038,#15039);
#12801=AXIS2_PLACEMENT_3D('',#18891,#15040,#15041);
#12802=AXIS2_PLACEMENT_3D('',#18893,#15042,#15043);
#12803=AXIS2_PLACEMENT_3D('',#18895,#15044,#15045);
#12804=AXIS2_PLACEMENT_3D('',#18897,#15046,#15047);
#12805=AXIS2_PLACEMENT_3D('',#18899,#15048,#15049);
#12806=AXIS2_PLACEMENT_3D('',#18901,#15050,#15051);
#12807=AXIS2_PLACEMENT_3D('',#18903,#15052,#15053);
#12808=AXIS2_PLACEMENT_3D('',#18905,#15054,#15055);
#12809=AXIS2_PLACEMENT_3D('',#18906,#15056,#15057);
#12810=AXIS2_PLACEMENT_3D('',#18907,#15058,#15059);
#12811=AXIS2_PLACEMENT_3D('',#18910,#15060,#15061);
#12812=AXIS2_PLACEMENT_3D('',#18912,#15062,#15063);
#12813=AXIS2_PLACEMENT_3D('',#18914,#15064,#15065);
#12814=AXIS2_PLACEMENT_3D('',#18915,#15066,#15067);
#12815=AXIS2_PLACEMENT_3D('',#18917,#15068,#15069);
#12816=AXIS2_PLACEMENT_3D('',#18919,#15070,#15071);
#12817=AXIS2_PLACEMENT_3D('',#18921,#15072,#15073);
#12818=AXIS2_PLACEMENT_3D('',#18923,#15074,#15075);
#12819=AXIS2_PLACEMENT_3D('',#18925,#15076,#15077);
#12820=AXIS2_PLACEMENT_3D('',#18927,#15078,#15079);
#12821=AXIS2_PLACEMENT_3D('',#18929,#15080,#15081);
#12822=AXIS2_PLACEMENT_3D('',#18931,#15082,#15083);
#12823=AXIS2_PLACEMENT_3D('',#18933,#15084,#15085);
#12824=AXIS2_PLACEMENT_3D('',#18935,#15086,#15087);
#12825=AXIS2_PLACEMENT_3D('',#18936,#15088,#15089);
#12826=AXIS2_PLACEMENT_3D('',#18938,#15090,#15091);
#12827=AXIS2_PLACEMENT_3D('',#18939,#15092,#15093);
#12828=AXIS2_PLACEMENT_3D('',#18941,#15095,#15096);
#12829=AXIS2_PLACEMENT_3D('',#18947,#15097,#15098);
#12830=AXIS2_PLACEMENT_3D('',#18951,#15099,#15100);
#12831=AXIS2_PLACEMENT_3D('',#18957,#15101,#15102);
#12832=AXIS2_PLACEMENT_3D('',#18961,#15103,#15104);
#12833=AXIS2_PLACEMENT_3D('',#18967,#15105,#15106);
#12834=AXIS2_PLACEMENT_3D('',#18971,#15107,#15108);
#12835=AXIS2_PLACEMENT_3D('',#18972,#15109,#15110);
#12836=AXIS2_PLACEMENT_3D('',#18978,#15111,#15112);
#12837=AXIS2_PLACEMENT_3D('',#18982,#15113,#15114);
#12838=AXIS2_PLACEMENT_3D('',#18986,#15116,#15117);
#12839=AXIS2_PLACEMENT_3D('',#18988,#15119,#15120);
#12840=AXIS2_PLACEMENT_3D('',#18993,#15122,#15123);
#12841=AXIS2_PLACEMENT_3D('',#18998,#15125,#15126);
#12842=AXIS2_PLACEMENT_3D('',#19005,#15129,#15130);
#12843=AXIS2_PLACEMENT_3D('',#19012,#15133,#15134);
#12844=AXIS2_PLACEMENT_3D('',#19013,#15135,#15136);
#12845=AXIS2_PLACEMENT_3D('',#19014,#15137,#15138);
#12846=AXIS2_PLACEMENT_3D('',#19017,#15141,#15142);
#12847=AXIS2_PLACEMENT_3D('',#19019,#15144,#15145);
#12848=AXIS2_PLACEMENT_3D('',#19021,#15147,#15148);
#12849=AXIS2_PLACEMENT_3D('',#19028,#15151,#15152);
#12850=AXIS2_PLACEMENT_3D('',#19035,#15155,#15156);
#12851=AXIS2_PLACEMENT_3D('',#19036,#15157,#15158);
#12852=AXIS2_PLACEMENT_3D('',#19037,#15159,#15160);
#12853=AXIS2_PLACEMENT_3D('',#19038,#15161,#15162);
#12854=AXIS2_PLACEMENT_3D('',#19039,#15163,#15164);
#12855=AXIS2_PLACEMENT_3D('',#19040,#15165,#15166);
#12856=AXIS2_PLACEMENT_3D('',#19041,#15167,#15168);
#12857=AXIS2_PLACEMENT_3D('',#19042,#15169,#15170);
#12858=AXIS2_PLACEMENT_3D('',#19043,#15171,#15172);
#15007=DIRECTION('axis',(0.,0.,1.));
#15008=DIRECTION('refdir',(1.,0.,0.));
#15009=DIRECTION('center_axis',(-0.0498412966806708,0.998757150234825,2.18495763504859E-17));
#15010=DIRECTION('ref_axis',(0.695179757024366,0.0346917771833739,0.717998318953048));
#15011=DIRECTION('center_axis',(-0.0498412966806708,0.998757150234825,2.18495763504859E-17));
#15012=DIRECTION('ref_axis',(0.695179757024367,0.034691777183374,0.717998318953046));
#15013=DIRECTION('center_axis',(-0.0498412966806708,0.998757150234825,2.18495763504859E-17));
#15014=DIRECTION('ref_axis',(0.695179757024367,0.034691777183374,0.717998318953046));
#15015=DIRECTION('',(0.526809439201579,-0.68169716279182,0.507701480212241));
#15016=DIRECTION('center_axis',(0.0498412966806708,-0.998757150234825,-2.18495763504859E-17));
#15017=DIRECTION('ref_axis',(0.69517975702437,0.0346917771833741,0.717998318953044));
#15018=DIRECTION('center_axis',(0.0498412966806708,-0.998757150234825,-2.18495763504859E-17));
#15019=DIRECTION('ref_axis',(-0.695179757024368,-0.034691777183374,-0.717998318953046));
#15020=DIRECTION('center_axis',(-0.0498412966806708,0.998757150234825,2.18495763504859E-17));
#15021=DIRECTION('ref_axis',(-0.695179757024368,-0.034691777183374,-0.717998318953046));
#15022=DIRECTION('center_axis',(0.0498412966806708,-0.998757150234825,-2.18495763504859E-17));
#15023=DIRECTION('ref_axis',(0.69517975702437,0.0346917771833741,0.717998318953044));
#15024=DIRECTION('center_axis',(0.695179757024367,0.0346917771833744,0.717998318953047));
#15025=DIRECTION('ref_axis',(0.71710595491094,0.0357859672311607,-0.696044836185572));
#15026=DIRECTION('center_axis',(-0.0498412966806708,0.998757150234825,2.18495763504859E-17));
#15027=DIRECTION('ref_axis',(-0.695179757024368,-0.034691777183374,-0.717998318953046));
#15028=DIRECTION('center_axis',(-0.526809439201581,0.681697162791818,-0.507701480212242));
#15029=DIRECTION('ref_axis',(-0.456323201469511,-0.730758744587374,-0.507701480212241));
#15030=DIRECTION('center_axis',(-0.0498412966806708,0.998757150234825,2.18495763504859E-17));
#15031=DIRECTION('ref_axis',(-0.695179757024366,-0.0346917771833739,-0.717998318953048));
#15032=DIRECTION('center_axis',(0.47182736468075,0.731532453790069,-0.492178023676697));
#15033=DIRECTION('ref_axis',(0.542313602412785,-0.680923453589126,-0.492178023676724));
#15034=DIRECTION('center_axis',(-0.0498412966806708,0.998757150234825,2.18495763504859E-17));
#15035=DIRECTION('ref_axis',(-0.695179757024368,-0.034691777183374,-0.717998318953046));
#15036=DIRECTION('center_axis',(-0.542313602412816,0.680923453589121,0.492178023676697));
#15037=DIRECTION('ref_axis',(0.471827364680741,0.731532453790072,-0.492178023676701));
#15038=DIRECTION('center_axis',(-0.0498412966806708,0.998757150234825,2.18495763504859E-17));
#15039=DIRECTION('ref_axis',(-0.695179757024374,-0.0346917771833743,-0.71799831895304));
#15040=DIRECTION('center_axis',(-0.526809439201581,0.681697162791818,-0.507701480212242));
#15041=DIRECTION('ref_axis',(-0.456323201469524,-0.730758744587375,-0.507701480212228));
#15042=DIRECTION('center_axis',(-0.0498412966806708,0.998757150234825,2.18495763504859E-17));
#15043=DIRECTION('ref_axis',(-0.695179757024368,-0.034691777183374,-0.717998318953046));
#15044=DIRECTION('center_axis',(0.456323201469515,0.730758744587371,0.507701480212242));
#15045=DIRECTION('ref_axis',(-0.526809439201585,0.681697162791821,-0.507701480212233));
#15046=DIRECTION('center_axis',(-0.0498412966806708,0.998757150234825,2.18495763504859E-17));
#15047=DIRECTION('ref_axis',(-0.695179757024363,-0.0346917771833738,-0.71799831895305));
#15048=DIRECTION('center_axis',(-0.542313602412816,0.680923453589121,0.492178023676697));
#15049=DIRECTION('ref_axis',(0.471827364680746,0.731532453790072,-0.492178023676696));
#15050=DIRECTION('center_axis',(-0.0498412966806708,0.998757150234825,2.18495763504859E-17));
#15051=DIRECTION('ref_axis',(-0.69517975702437,-0.0346917771833741,-0.717998318953044));
#15052=DIRECTION('center_axis',(0.47182736468075,0.731532453790069,-0.492178023676697));
#15053=DIRECTION('ref_axis',(0.542313602412809,-0.680923453589124,-0.492178023676699));
#15054=DIRECTION('center_axis',(-0.0498412966806708,0.998757150234825,2.18495763504859E-17));
#15055=DIRECTION('ref_axis',(-0.695179757024366,-0.0346917771833739,-0.717998318953048));
#15056=DIRECTION('center_axis',(0.456323201469515,0.730758744587371,0.507701480212242));
#15057=DIRECTION('ref_axis',(-0.526809439201583,0.681697162791821,-0.507701480212235));
#15058=DIRECTION('center_axis',(-0.695179757024368,-0.0346917771833739,
-0.717998318953046));
#15059=DIRECTION('ref_axis',(-0.71710595491094,-0.0357859672311622,0.696044836185572));
#15060=DIRECTION('center_axis',(0.0498412966806708,-0.998757150234825,-2.18495763504859E-17));
#15061=DIRECTION('ref_axis',(0.695179757024368,0.034691777183374,0.717998318953046));
#15062=DIRECTION('center_axis',(-0.456323201469515,-0.730758744587371,-0.507701480212242));
#15063=DIRECTION('ref_axis',(-0.526809439201578,0.681697162791822,-0.50770148021224));
#15064=DIRECTION('center_axis',(0.0498412966806708,-0.998757150234825,-2.18495763504859E-17));
#15065=DIRECTION('ref_axis',(-0.695179757024368,-0.034691777183374,-0.717998318953046));
#15066=DIRECTION('center_axis',(-0.47182736468075,-0.731532453790069,0.492178023676697));
#15067=DIRECTION('ref_axis',(0.542313602412811,-0.680923453589124,-0.492178023676697));
#15068=DIRECTION('center_axis',(0.542313602412816,-0.680923453589121,-0.492178023676697));
#15069=DIRECTION('ref_axis',(0.471827364680746,0.731532453790072,-0.492178023676696));
#15070=DIRECTION('center_axis',(0.0498412966806708,-0.998757150234825,-2.18495763504859E-17));
#15071=DIRECTION('ref_axis',(-0.695179757024368,-0.034691777183374,-0.717998318953046));
#15072=DIRECTION('center_axis',(-0.456323201469515,-0.730758744587371,-0.507701480212242));
#15073=DIRECTION('ref_axis',(-0.526809439201578,0.681697162791822,-0.50770148021224));
#15074=DIRECTION('center_axis',(0.0498412966806708,-0.998757150234825,-2.18495763504859E-17));
#15075=DIRECTION('ref_axis',(0.695179757024362,0.0346917771833737,0.717998318953052));
#15076=DIRECTION('center_axis',(0.526809439201581,-0.681697162791818,0.507701480212242));
#15077=DIRECTION('ref_axis',(-0.456323201469513,-0.730758744587375,-0.507701480212239));
#15078=DIRECTION('center_axis',(0.0498412966806708,-0.998757150234825,-2.18495763504859E-17));
#15079=DIRECTION('ref_axis',(-0.695179757024368,-0.034691777183374,-0.717998318953046));
#15080=DIRECTION('center_axis',(0.542313602412816,-0.680923453589121,-0.492178023676697));
#15081=DIRECTION('ref_axis',(0.471827364680746,0.731532453790072,-0.492178023676696));
#15082=DIRECTION('center_axis',(0.0498412966806708,-0.998757150234825,-2.18495763504859E-17));
#15083=DIRECTION('ref_axis',(0.695179757024367,0.034691777183374,0.717998318953047));
#15084=DIRECTION('center_axis',(-0.47182736468075,-0.731532453790069,0.492178023676697));
#15085=DIRECTION('ref_axis',(0.542313602412811,-0.680923453589124,-0.492178023676697));
#15086=DIRECTION('center_axis',(0.0498412966806708,-0.998757150234825,-2.18495763504859E-17));
#15087=DIRECTION('ref_axis',(-0.695179757024368,-0.034691777183374,-0.717998318953046));
#15088=DIRECTION('center_axis',(0.526809439201581,-0.681697162791818,0.507701480212242));
#15089=DIRECTION('ref_axis',(-0.456323201469513,-0.730758744587375,-0.507701480212239));
#15090=DIRECTION('center_axis',(0.0498412966806708,-0.998757150234825,-2.18495763504859E-17));
#15091=DIRECTION('ref_axis',(-0.695179757024367,-0.034691777183374,-0.717998318953046));
#15092=DIRECTION('center_axis',(0.0498412966806708,-0.998757150234825,-2.18495763504859E-17));
#15093=DIRECTION('ref_axis',(-0.695179757024367,-0.034691777183374,-0.717998318953046));
#15094=DIRECTION('',(-0.0498412966806708,0.998757150234825,2.18495763504859E-17));
#15095=DIRECTION('center_axis',(0.0498412966806708,-0.998757150234825,-2.18495763504859E-17));
#15096=DIRECTION('ref_axis',(-0.695179757024367,-0.034691777183374,-0.717998318953047));
#15097=DIRECTION('center_axis',(0.0498412966806708,-0.998757150234825,-2.18495763504859E-17));
#15098=DIRECTION('ref_axis',(-0.695179757024368,-0.034691777183374,-0.717998318953046));
#15099=DIRECTION('center_axis',(0.0498412966806708,-0.998757150234825,-2.18495763504859E-17));
#15100=DIRECTION('ref_axis',(-0.695179757024367,-0.034691777183374,-0.717998318953047));
#15101=DIRECTION('center_axis',(0.0498412966806708,-0.998757150234825,-2.18495763504859E-17));
#15102=DIRECTION('ref_axis',(-0.695179757024368,-0.034691777183374,-0.717998318953046));
#15103=DIRECTION('center_axis',(0.0498412966806708,-0.998757150234825,-2.18495763504859E-17));
#15104=DIRECTION('ref_axis',(-0.695179757024367,-0.034691777183374,-0.717998318953047));
#15105=DIRECTION('center_axis',(0.0498412966806708,-0.998757150234825,-2.18495763504859E-17));
#15106=DIRECTION('ref_axis',(-0.695179757024368,-0.034691777183374,-0.717998318953046));
#15107=DIRECTION('center_axis',(-0.0498412966806708,0.998757150234825,1.38777878078145E-17));
#15108=DIRECTION('ref_axis',(0.695179757024368,0.034691777183374,0.717998318953046));
#15109=DIRECTION('center_axis',(0.0498412966806708,-0.998757150234825,-2.18495763504859E-17));
#15110=DIRECTION('ref_axis',(-0.695179757024367,-0.034691777183374,-0.717998318953047));
#15111=DIRECTION('center_axis',(0.0498412966806708,-0.998757150234825,-2.18495763504859E-17));
#15112=DIRECTION('ref_axis',(-0.695179757024368,-0.034691777183374,-0.717998318953046));
#15113=DIRECTION('center_axis',(0.0498412966806708,-0.998757150234825,-1.38777878078145E-17));
#15114=DIRECTION('ref_axis',(-0.695179757024368,-0.034691777183374,-0.717998318953046));
#15115=DIRECTION('',(0.71710595491094,0.0357859672311617,-0.696044836185572));
#15116=DIRECTION('center_axis',(-0.0498412966806708,0.998757150234825,2.18495763504859E-17));
#15117=DIRECTION('ref_axis',(-0.695179757024367,-0.034691777183374,-0.717998318953047));
#15118=DIRECTION('',(0.71710595491094,0.0357859672311617,-0.696044836185572));
#15119=DIRECTION('center_axis',(-0.456323201469515,-0.730758744587371,-0.507701480212242));
#15120=DIRECTION('ref_axis',(-0.526809439201578,0.681697162791822,-0.507701480212239));
#15121=DIRECTION('',(-0.71710595491094,-0.0357859672311617,0.696044836185572));
#15122=DIRECTION('center_axis',(0.526809439201581,-0.681697162791818,0.507701480212242));
#15123=DIRECTION('ref_axis',(-0.456323201469513,-0.730758744587375,-0.507701480212239));
#15124=DIRECTION('',(0.71710595491094,0.0357859672311617,-0.696044836185572));
#15125=DIRECTION('center_axis',(0.526809439201581,-0.681697162791818,0.507701480212242));
#15126=DIRECTION('ref_axis',(-0.456323201469513,-0.730758744587375,-0.507701480212239));
#15127=DIRECTION('',(0.71710595491094,0.0357859672311617,-0.696044836185572));
#15128=DIRECTION('',(0.71710595491094,0.0357859672311617,-0.696044836185572));
#15129=DIRECTION('center_axis',(-0.456323201469515,-0.730758744587371,-0.507701480212242));
#15130=DIRECTION('ref_axis',(-0.526809439201578,0.681697162791822,-0.507701480212239));
#15131=DIRECTION('',(-0.71710595491094,-0.0357859672311617,0.696044836185572));
#15132=DIRECTION('',(0.71710595491094,0.0357859672311617,-0.696044836185572));
#15133=DIRECTION('center_axis',(0.0498412966806708,-0.998757150234825,-1.38777878078145E-17));
#15134=DIRECTION('ref_axis',(-0.695179757024368,-0.034691777183374,-0.717998318953046));
#15135=DIRECTION('center_axis',(-0.0498412966806708,0.998757150234825,2.18495763504859E-17));
#15136=DIRECTION('ref_axis',(-0.695179757024368,-0.034691777183374,-0.717998318953046));
#15137=DIRECTION('center_axis',(0.0498412966806708,-0.998757150234825,-1.38777878078145E-17));
#15138=DIRECTION('ref_axis',(-0.695179757024368,-0.034691777183374,-0.717998318953046));
#15139=DIRECTION('',(0.695179757024365,0.0346917771833739,0.717998318953049));
#15140=DIRECTION('',(0.695179757024365,0.0346917771833739,0.717998318953049));
#15141=DIRECTION('center_axis',(0.542313602412816,-0.68092345358912,-0.492178023676697));
#15142=DIRECTION('ref_axis',(0.471827364680746,0.731532453790072,-0.492178023676696));
#15143=DIRECTION('',(-0.695179757024365,-0.0346917771833739,-0.717998318953049));
#15144=DIRECTION('center_axis',(-0.47182736468075,-0.731532453790069,0.492178023676697));
#15145=DIRECTION('ref_axis',(0.542313602412812,-0.680923453589124,-0.492178023676696));
#15146=DIRECTION('',(0.695179757024365,0.0346917771833739,0.717998318953049));
#15147=DIRECTION('center_axis',(-0.47182736468075,-0.731532453790069,0.492178023676697));
#15148=DIRECTION('ref_axis',(0.542313602412812,-0.680923453589124,-0.492178023676696));
#15149=DIRECTION('',(0.695179757024365,0.0346917771833739,0.717998318953049));
#15150=DIRECTION('',(0.695179757024365,0.0346917771833739,0.717998318953049));
#15151=DIRECTION('center_axis',(0.542313602412816,-0.68092345358912,-0.492178023676697));
#15152=DIRECTION('ref_axis',(0.471827364680746,0.731532453790072,-0.492178023676696));
#15153=DIRECTION('',(-0.695179757024365,-0.0346917771833739,-0.717998318953049));
#15154=DIRECTION('',(0.695179757024365,0.0346917771833739,0.717998318953049));
#15155=DIRECTION('center_axis',(0.0498412966806708,-0.998757150234825,-1.38777878078145E-17));
#15156=DIRECTION('ref_axis',(-0.695179757024368,-0.034691777183374,-0.717998318953046));
#15157=DIRECTION('center_axis',(-0.0498412966806708,0.998757150234825,2.18495763504859E-17));
#15158=DIRECTION('ref_axis',(-0.695179757024368,-0.034691777183374,-0.717998318953046));
#15159=DIRECTION('center_axis',(0.0498412966806708,-0.998757150234825,-1.04083408558608E-17));
#15160=DIRECTION('ref_axis',(-0.695179757024368,-0.034691777183374,-0.717998318953046));
#15161=DIRECTION('center_axis',(0.0498412966806708,-0.998757150234825,-1.04083408558608E-17));
#15162=DIRECTION('ref_axis',(-0.695179757024368,-0.034691777183374,-0.717998318953046));
#15163=DIRECTION('center_axis',(0.0498412966806708,-0.998757150234825,-1.04083408558608E-17));
#15164=DIRECTION('ref_axis',(-0.695179757024368,-0.034691777183374,-0.717998318953046));
#15165=DIRECTION('center_axis',(0.0498412966806708,-0.998757150234825,-1.04083408558608E-17));
#15166=DIRECTION('ref_axis',(-0.695179757024368,-0.034691777183374,-0.717998318953046));
#15167=DIRECTION('center_axis',(0.0498412966806708,-0.998757150234825,-2.18495763504859E-17));
#15168=DIRECTION('ref_axis',(-0.695179757024368,-0.034691777183374,-0.717998318953046));
#15169=DIRECTION('center_axis',(0.0498412966806708,-0.998757150234825,-2.18495763504859E-17));
#15170=DIRECTION('ref_axis',(0.695179757024366,0.0346917771833739,0.717998318953047));
#15171=DIRECTION('center_axis',(0.0498412966806708,-0.998757150234825,-2.18495763504859E-17));
#15172=DIRECTION('ref_axis',(-0.695179757024368,-0.034691777183374,-0.717998318953046));
#18852=CARTESIAN_POINT('',(0.,0.,0.));
#18853=CARTESIAN_POINT('Origin',(-231.689233855248,191.349200530894,253.073593133704));
#18854=CARTESIAN_POINT('',(-223.099169485805,193.780362046156,262.048572120617));
#18855=CARTESIAN_POINT('',(-240.478663411414,192.913067616571,244.098614146791));
#18856=CARTESIAN_POINT('Origin',(-231.78891644861,193.346714831364,253.073593133704));
#18857=CARTESIAN_POINT('Origin',(-231.78891644861,193.346714831364,253.073593133704));
#18858=CARTESIAN_POINT('',(-238.988621304004,190.984936870468,245.534610784697));
#18859=CARTESIAN_POINT('',(-238.988621304004,190.984936870468,245.534610784697));
#18860=CARTESIAN_POINT('Origin',(-231.689233855248,191.349200530894,253.073593133704));
#18861=CARTESIAN_POINT('Origin',(-237.419514171664,306.176839858541,253.073593133704));
#18862=CARTESIAN_POINT('',(-250.440271285438,306.057676646063,218.820732405352));
#18863=CARTESIAN_POINT('',(-271.236343977855,305.019883596359,239.006032654733));
#18864=CARTESIAN_POINT('Origin',(-237.44592788123,306.706137510275,253.073593133704));
#18865=CARTESIAN_POINT('',(-251.347266456762,305.48179879318,218.618067764708));
#18866=CARTESIAN_POINT('Ctrl Pts',(-251.347266456762,305.48179879318,218.618067764708));
#18867=CARTESIAN_POINT('Ctrl Pts',(-250.891701988272,305.772942264292,218.717244054283));
#18868=CARTESIAN_POINT('Ctrl Pts',(-250.440271285437,306.057676646063,218.820732405352));
#18869=CARTESIAN_POINT('',(-271.383269500837,304.481935741607,238.065621311184));
#18870=CARTESIAN_POINT('Origin',(-237.419514171664,306.176839858541,253.073593133704));
#18871=CARTESIAN_POINT('Ctrl Pts',(-271.236343977855,305.019883596359,239.006032654733));
#18872=CARTESIAN_POINT('Ctrl Pts',(-271.312182393571,304.75389251631,238.537983013705));
#18873=CARTESIAN_POINT('Ctrl Pts',(-271.383269500837,304.481935741607,238.065621311184));
#18874=CARTESIAN_POINT('Origin',(-239.027345521937,338.395766018202,253.073593133704));
#18875=CARTESIAN_POINT('',(-264.591821718871,305.351467310312,259.227189433814));
#18876=CARTESIAN_POINT('',(-244.431608765165,306.35752884863,280.049140683453));
#18877=CARTESIAN_POINT('Origin',(-237.44592788123,306.706137510275,253.073593133704));
#18878=CARTESIAN_POINT('',(-243.894079636939,308.886976989217,282.887702827629));
#18879=CARTESIAN_POINT('Origin',(-221.806532920431,316.111846600949,269.669787882023));
#18880=CARTESIAN_POINT('',(-232.174356018737,309.471830095633,283.069881793484));
#18881=CARTESIAN_POINT('Origin',(-237.570506863568,309.202544258603,253.073593133704));
#18882=CARTESIAN_POINT('',(-231.299979576836,307.012840729122,280.253267222905));
#18883=CARTESIAN_POINT('Origin',(-254.450855472222,314.482786558815,269.162343413428));
#18884=CARTESIAN_POINT('',(-210.503906884418,308.050633778826,260.067966973523));
#18885=CARTESIAN_POINT('Origin',(-237.44592788123,306.706137510275,253.073593133704));
#18886=CARTESIAN_POINT('',(-207.793451628875,310.688518145128,259.405034938035));
#18887=CARTESIAN_POINT('Origin',(-221.299719129075,316.137138291257,236.984842853979));
#18888=CARTESIAN_POINT('',(-207.611499084105,310.697598181014,247.670727338388));
#18889=CARTESIAN_POINT('Origin',(-237.570506863568,309.202544258603,253.073593133704));
#18890=CARTESIAN_POINT('',(-210.300034043588,308.060807710239,246.919996833593));
#18891=CARTESIAN_POINT('Origin',(-221.806532920431,316.111846600949,269.669787882023));
#18892=CARTESIAN_POINT('',(-230.460246997295,307.054746171921,226.098045583955));
#18893=CARTESIAN_POINT('Origin',(-237.44592788123,306.706137510275,253.073593133704));
#18894=CARTESIAN_POINT('',(-231.246934090196,309.518111527989,223.259483439779));
#18895=CARTESIAN_POINT('Origin',(-253.944041680866,314.508078249123,236.477398385385));
#18896=CARTESIAN_POINT('',(-242.966657708398,308.933258421573,223.077304473924));
#18897=CARTESIAN_POINT('Origin',(-237.570506863568,309.202544258603,253.073593133704));
#18898=CARTESIAN_POINT('',(-243.591876185624,306.399434291429,225.893919044503));
#18899=CARTESIAN_POINT('Origin',(-221.299719129075,316.137138291257,236.984842853979));
#18900=CARTESIAN_POINT('',(-264.387948878041,305.361641241725,246.079219293884));
#18901=CARTESIAN_POINT('Origin',(-237.44592788123,306.706137510275,253.073593133704));
#18902=CARTESIAN_POINT('',(-267.347562098261,307.716570372078,246.742151329373));
#18903=CARTESIAN_POINT('Origin',(-254.450855472222,314.482786558815,269.162343413428));
#18904=CARTESIAN_POINT('',(-267.52951464303,307.707490336192,258.47645892902));
#18905=CARTESIAN_POINT('Origin',(-237.570506863568,309.202544258603,253.073593133704));
#18906=CARTESIAN_POINT('Origin',(-253.944041680866,314.508078249123,236.477398385385));
#18907=CARTESIAN_POINT('Origin',(-239.086294923286,339.57703817644,253.073593133704));
#18908=CARTESIAN_POINT('',(-252.408833339929,305.42882308236,287.079612836479));
#18909=CARTESIAN_POINT('',(-271.832216499046,304.459531796337,267.018677063088));
#18910=CARTESIAN_POINT('Origin',(-237.419514171664,306.176839858541,253.073593133704));
#18911=CARTESIAN_POINT('',(-272.435152125237,304.96005909095,266.840164323315));
#18912=CARTESIAN_POINT('Origin',(-254.384625574476,315.07819861504,236.052794955191));
#18913=CARTESIAN_POINT('',(-271.991461983488,304.982200701635,238.226128675688));
#18914=CARTESIAN_POINT('Origin',(-237.44592788123,306.706137510275,253.073593133704));
#18915=CARTESIAN_POINT('Origin',(-254.904405884816,315.052259852398,269.573964189148));
#18916=CARTESIAN_POINT('',(-251.19538929107,306.019993751338,218.040828426306));
#18917=CARTESIAN_POINT('Origin',(-220.905118117829,316.748937155912,236.573222078259));
#18918=CARTESIAN_POINT('',(-222.616916590929,307.446154391283,218.485070694454));
#18919=CARTESIAN_POINT('Origin',(-237.44592788123,306.706137510275,253.073593133704));
#18920=CARTESIAN_POINT('',(-222.4301950034,306.924856634723,219.067573430929));
#18921=CARTESIAN_POINT('Origin',(-254.384625574476,315.07819861504,236.052794955191));
#18922=CARTESIAN_POINT('',(-203.006811844283,307.894147920746,239.128509204319));
#18923=CARTESIAN_POINT('Origin',(-237.419514171664,306.176839858541,253.073593133704));
#18924=CARTESIAN_POINT('',(-202.456703637222,308.452215929601,239.307021944093));
#18925=CARTESIAN_POINT('Origin',(-221.42489842817,316.722998393271,270.094391312217));
#18926=CARTESIAN_POINT('',(-202.900393778972,308.430074318916,267.92105759172));
#18927=CARTESIAN_POINT('Origin',(-237.44592788123,306.706137510275,253.073593133704));
#18928=CARTESIAN_POINT('',(-203.455758842492,307.871743975476,268.081564956224));
#18929=CARTESIAN_POINT('Origin',(-220.905118117829,316.748937155912,236.573222078259));
#18930=CARTESIAN_POINT('',(-223.491761886567,306.871880923903,287.529118502699));
#18931=CARTESIAN_POINT('Origin',(-237.419514171664,306.176839858541,253.073593133704));
#18932=CARTESIAN_POINT('',(-223.696466471389,307.392281269213,288.106357841101));
#18933=CARTESIAN_POINT('Origin',(-254.904405884816,315.052259852398,269.573964189148));
#18934=CARTESIAN_POINT('',(-252.27493917153,305.966120629268,287.662115572953));
#18935=CARTESIAN_POINT('Origin',(-237.44592788123,306.706137510275,253.073593133704));
#18936=CARTESIAN_POINT('Origin',(-221.42489842817,316.722998393271,270.094391312217));
#18937=CARTESIAN_POINT('',(-227.983616560511,291.658562769169,262.048572120617));
#18938=CARTESIAN_POINT('Origin',(-236.673363523316,291.224915554376,253.073593133704));
#18939=CARTESIAN_POINT('Origin',(-231.689233855248,191.349200530894,253.073593133704));
#18940=CARTESIAN_POINT('',(-222.999486892444,191.782847745686,262.048572120617));
#18941=CARTESIAN_POINT('Origin',(-237.670189456929,311.200058559073,253.073593133704));
#18942=CARTESIAN_POINT('',(-228.761753229824,309.64213030126,286.594499765937));
#18943=CARTESIAN_POINT('Ctrl Pts',(-223.69646647139,307.392281269213,288.106357841101));
#18944=CARTESIAN_POINT('Ctrl Pts',(-226.31000387672,308.600428762359,287.396575304205));
#18945=CARTESIAN_POINT('Ctrl Pts',(-228.761753229824,309.64213030126,286.594499765937));
#18946=CARTESIAN_POINT('',(-247.414317038773,308.711305459166,286.304552247041));
#18947=CARTESIAN_POINT('Origin',(-237.570506863568,309.202544258603,253.073593133704));
#18948=CARTESIAN_POINT('Ctrl Pts',(-247.414317038773,308.711305459166,286.304552247041));
#18949=CARTESIAN_POINT('Ctrl Pts',(-249.773889204424,307.429503007661,287.031837490994));
#18950=CARTESIAN_POINT('Ctrl Pts',(-252.274939171527,305.96612062927,287.662115572952));
#18951=CARTESIAN_POINT('Origin',(-237.670189456929,311.200058559073,253.073593133704));
#18952=CARTESIAN_POINT('',(-271.049752044865,307.531818806141,261.893308348431));
#18953=CARTESIAN_POINT('Ctrl Pts',(-272.435152125237,304.96005909095,266.840164323315));
#18954=CARTESIAN_POINT('Ctrl Pts',(-271.792884971683,306.33068203763,264.290090789975));
#18955=CARTESIAN_POINT('Ctrl Pts',(-271.049752044865,307.531818806141,261.893308348431));
#18956=CARTESIAN_POINT('',(-270.760164887174,307.546270166452,243.217533356919));
#18957=CARTESIAN_POINT('Origin',(-237.570506863568,309.202544258603,253.073593133704));
#18958=CARTESIAN_POINT('Ctrl Pts',(-270.760164887174,307.546270166452,243.217533356919));
#18959=CARTESIAN_POINT('Ctrl Pts',(-271.428600472778,306.348861043188,240.797007088707));
#18960=CARTESIAN_POINT('Ctrl Pts',(-271.991461983488,304.982200701635,238.226128675688));
#18961=CARTESIAN_POINT('Origin',(-237.670189456929,311.200058559073,253.073593133704));
#18962=CARTESIAN_POINT('',(-204.09126168227,310.873269711066,244.253877918976));
#18963=CARTESIAN_POINT('Ctrl Pts',(-202.456703637222,308.452215929601,239.307021944093));
#18964=CARTESIAN_POINT('Ctrl Pts',(-203.232237251341,309.75208591228,241.857095477433));
#18965=CARTESIAN_POINT('Ctrl Pts',(-204.09126168227,310.873269711065,244.253877918976));
#18966=CARTESIAN_POINT('',(-204.380848839961,310.858818350754,262.929652910489));
#18967=CARTESIAN_POINT('Origin',(-237.570506863568,309.202544258603,253.073593133704));
#18968=CARTESIAN_POINT('Ctrl Pts',(-204.380848839961,310.858818350754,262.929652910489));
#18969=CARTESIAN_POINT('Ctrl Pts',(-203.596521750247,309.733906906721,265.350179178701));
#18970=CARTESIAN_POINT('Ctrl Pts',(-202.900393778972,308.430074318916,267.92105759172));
#18971=CARTESIAN_POINT('Origin',(-231.689233855248,191.349200530894,253.073593133704));
#18972=CARTESIAN_POINT('Origin',(-237.670189456929,311.200058559073,253.073593133704));
#18973=CARTESIAN_POINT('',(-246.379260497312,308.762958215947,219.55268650147));
#18974=CARTESIAN_POINT('Ctrl Pts',(-251.195389291067,306.019993751341,218.040828426307));
#18975=CARTESIAN_POINT('Ctrl Pts',(-248.715118346303,307.482339187552,218.750610963203));
#18976=CARTESIAN_POINT('Ctrl Pts',(-246.379260497312,308.762958215947,219.55268650147));
#18977=CARTESIAN_POINT('',(-227.726696688362,309.69378305804,219.842634020367));
#18978=CARTESIAN_POINT('Origin',(-237.570506863568,309.202544258603,253.073593133704));
#18979=CARTESIAN_POINT('Ctrl Pts',(-227.726696688362,309.69378305804,219.842634020367));
#18980=CARTESIAN_POINT('Ctrl Pts',(-225.251233018599,308.65326494225,219.115348776413));
#18981=CARTESIAN_POINT('Ctrl Pts',(-222.61691659093,307.446154391284,218.485070694455));
#18982=CARTESIAN_POINT('Origin',(-254.358103779067,305.86216380131,289.684098458565));
#18983=CARTESIAN_POINT('',(-203.23563831279,308.413344503999,240.063079615825));
#18984=CARTESIAN_POINT('',(-254.358103779067,305.86216380131,289.684098458565));
#18985=CARTESIAN_POINT('',(-223.395851266497,307.407282965681,219.241128366186));
#18986=CARTESIAN_POINT('Origin',(-237.44592788123,306.706137510275,253.073593133704));
#18987=CARTESIAN_POINT('',(-274.518316732773,304.856102262992,268.862147208927));
#18988=CARTESIAN_POINT('Origin',(-274.518316732773,304.856102262992,268.862147208927));
#18989=CARTESIAN_POINT('',(-276.380506741304,307.265796453966,267.067500884441));
#18990=CARTESIAN_POINT('Ctrl Pts',(-223.395851266497,307.407282965681,219.241128366186));
#18991=CARTESIAN_POINT('Ctrl Pts',(-222.915330871771,307.169056036833,219.152126865893));
#18992=CARTESIAN_POINT('Ctrl Pts',(-222.4301950034,306.924856634723,219.067573430929));
#18993=CARTESIAN_POINT('Origin',(-251.454394814525,310.512180961828,292.914741420956));
#18994=CARTESIAN_POINT('',(-252.745071735212,308.445283106991,291.47874478305));
#18995=CARTESIAN_POINT('Ctrl Pts',(-203.006811844283,307.894147920746,239.128509204319));
#18996=CARTESIAN_POINT('Ctrl Pts',(-203.11922611311,308.156947367739,239.598018442737));
#18997=CARTESIAN_POINT('Ctrl Pts',(-203.23563831279,308.413344503999,240.063079615825));
#18998=CARTESIAN_POINT('Origin',(-251.454394814525,310.512180961828,292.914741420956));
#18999=CARTESIAN_POINT('',(-252.745071735212,308.445283106991,291.47874478305));
#19000=CARTESIAN_POINT('',(-251.496004495962,306.00499205487,286.906057901221));
#19001=CARTESIAN_POINT('',(-254.358103779067,305.86216380131,289.684098458565));
#19002=CARTESIAN_POINT('Ctrl Pts',(-251.496004495962,306.00499205487,286.906057901221));
#19003=CARTESIAN_POINT('Ctrl Pts',(-251.950419952519,305.720108723982,286.995059401515));
#19004=CARTESIAN_POINT('Ctrl Pts',(-252.408833339929,305.42882308236,287.079612836479));
#19005=CARTESIAN_POINT('Origin',(-274.518316732773,304.856102262992,268.862147208927));
#19006=CARTESIAN_POINT('',(-276.380506741304,307.265796453966,267.067500884441));
#19007=CARTESIAN_POINT('',(-271.656217449669,304.998930516552,266.084106651583));
#19008=CARTESIAN_POINT('Ctrl Pts',(-271.832216499046,304.459531796337,267.018677063088));
#19009=CARTESIAN_POINT('Ctrl Pts',(-271.746524711181,304.732217393075,266.549167824671));
#19010=CARTESIAN_POINT('Ctrl Pts',(-271.656217449669,304.998930516552,266.084106651583));
#19011=CARTESIAN_POINT('',(-274.518316732773,304.856102262992,268.862147208927));
#19012=CARTESIAN_POINT('Origin',(-254.358103779067,305.86216380131,289.684098458565));
#19013=CARTESIAN_POINT('Origin',(-237.44592788123,306.706137510275,253.073593133704));
#19014=CARTESIAN_POINT('Origin',(-274.010931848145,304.88142245275,236.14037178569));
#19015=CARTESIAN_POINT('',(-253.214859155728,305.919215502453,215.955071536309));
#19016=CARTESIAN_POINT('',(-274.010931848145,304.88142245275,236.14037178569));
#19017=CARTESIAN_POINT('Origin',(-253.214859155728,305.919215502453,215.955071536309));
#19018=CARTESIAN_POINT('',(-251.547022289343,308.505069750677,214.215298233275));
#19019=CARTESIAN_POINT('Origin',(-277.461821182389,309.214324067189,239.272234761095));
#19020=CARTESIAN_POINT('',(-275.927926679205,307.288381701182,237.880145088724));
#19021=CARTESIAN_POINT('Origin',(-277.461821182389,309.214324067189,239.272234761095));
#19022=CARTESIAN_POINT('',(-275.927926679205,307.288381701182,237.880145088724));
#19023=CARTESIAN_POINT('',(-224.451584477021,307.354598374488,287.326453862056));
#19024=CARTESIAN_POINT('Ctrl Pts',(-223.491761886567,306.871880923903,287.529118502699));
#19025=CARTESIAN_POINT('Ctrl Pts',(-223.974048836019,307.116222496522,287.429942213125));
#19026=CARTESIAN_POINT('Ctrl Pts',(-224.451584477021,307.354598374488,287.326453862056));
#19027=CARTESIAN_POINT('',(-274.010931848145,304.88142245275,236.14037178569));
#19028=CARTESIAN_POINT('Origin',(-253.214859155728,305.919215502453,215.955071536309));
#19029=CARTESIAN_POINT('',(-251.547022289343,308.505069750677,214.215298233275));
#19030=CARTESIAN_POINT('',(-203.655511784604,308.392391424192,267.141153612674));
#19031=CARTESIAN_POINT('',(-253.214859155728,305.919215502453,215.955071536309));
#19032=CARTESIAN_POINT('Ctrl Pts',(-203.655511784604,308.392391424192,267.141153612674));
#19033=CARTESIAN_POINT('Ctrl Pts',(-203.55356843072,308.135272244505,267.609203253702));
#19034=CARTESIAN_POINT('Ctrl Pts',(-203.455758842491,307.871743975476,268.081564956224));
#19035=CARTESIAN_POINT('Origin',(-274.010931848145,304.88142245275,236.14037178569));
#19036=CARTESIAN_POINT('Origin',(-237.44592788123,306.706137510275,253.073593133704));
#19037=CARTESIAN_POINT('Origin',(-240.071393924063,309.077741693818,304.568423058936));
#19038=CARTESIAN_POINT('Origin',(-240.071393924063,309.077741693818,304.568423058936));
#19039=CARTESIAN_POINT('Origin',(-240.071393924063,309.077741693818,304.568423058936));
#19040=CARTESIAN_POINT('Origin',(-240.071393924063,309.077741693818,304.568423058936));
#19041=CARTESIAN_POINT('Origin',(-237.419514171664,306.176839858541,253.073593133704));
#19042=CARTESIAN_POINT('Origin',(-237.419514171664,306.176839858541,253.073593133704));
#19043=CARTESIAN_POINT('Origin',(-237.419514171664,306.176839858541,253.073593133704));
#27756=UNCERTAINTY_MEASURE_WITH_UNIT(LENGTH_MEASURE(0.01),#27808,
'DISTANCE_ACCURACY_VALUE',
'Maximum model space distance between geometric entities at asserted c
onnectivities');
#27778=UNCERTAINTY_MEASURE_WITH_UNIT(LENGTH_MEASURE(0.01),#27808,
'DISTANCE_ACCURACY_VALUE',
'Maximum model space distance between geometric entities at asserted c
onnectivities');
#27785=(
GEOMETRIC_REPRESENTATION_CONTEXT(3)
GLOBAL_UNCERTAINTY_ASSIGNED_CONTEXT((#27756))
GLOBAL_UNIT_ASSIGNED_CONTEXT((#27808,#27810,#27811))
REPRESENTATION_CONTEXT('','3D')
);
#27807=(
GEOMETRIC_REPRESENTATION_CONTEXT(3)
GLOBAL_UNCERTAINTY_ASSIGNED_CONTEXT((#27778))
GLOBAL_UNIT_ASSIGNED_CONTEXT((#27808,#27810,#27811))
REPRESENTATION_CONTEXT('','3D')
);
#27808=(
LENGTH_UNIT()
NAMED_UNIT(*)
SI_UNIT(.MILLI.,.METRE.)
);
#27810=(
NAMED_UNIT(*)
PLANE_ANGLE_UNIT()
SI_UNIT($,.RADIAN.)
);
#27811=(
NAMED_UNIT(*)
SI_UNIT($,.STERADIAN.)
SOLID_ANGLE_UNIT()
);
#27818=SHAPE_DEFINITION_REPRESENTATION(#27848,#27905);
#27848=PRODUCT_DEFINITION_SHAPE('',$,#27934);
#27905=SHAPE_REPRESENTATION('',(#12785),#27785);
#27927=PRODUCT_DEFINITION_CONTEXT('part definition',#28013,'design');
#27934=PRODUCT_DEFINITION('Lifting Saddle','Lifting Saddle',#27962,#27927);
#27962=PRODUCT_DEFINITION_FORMATION('',$,#28021);
#28013=APPLICATION_CONTEXT('Managed model based 3d engineering');
#28014=PRODUCT_CONTEXT('part definition',#28013,'mechanical');
#28021=PRODUCT('Lifting Saddle','Lifting Saddle',$,(#28014));
#28064=COLOUR_RGB('Sky Blue',0.24,0.69,0.87);
#28065=FILL_AREA_STYLE_COLOUR('',#28064);
#28066=FILL_AREA_STYLE('',(#28065));
#28067=SURFACE_STYLE_FILL_AREA(#28066);
#28068=SURFACE_SIDE_STYLE('',(#28067));
#28069=SURFACE_STYLE_USAGE(.BOTH.,#28068);
#28070=PRESENTATION_STYLE_ASSIGNMENT((#28069));
ENDSEC;
END-ISO-10303-21;
